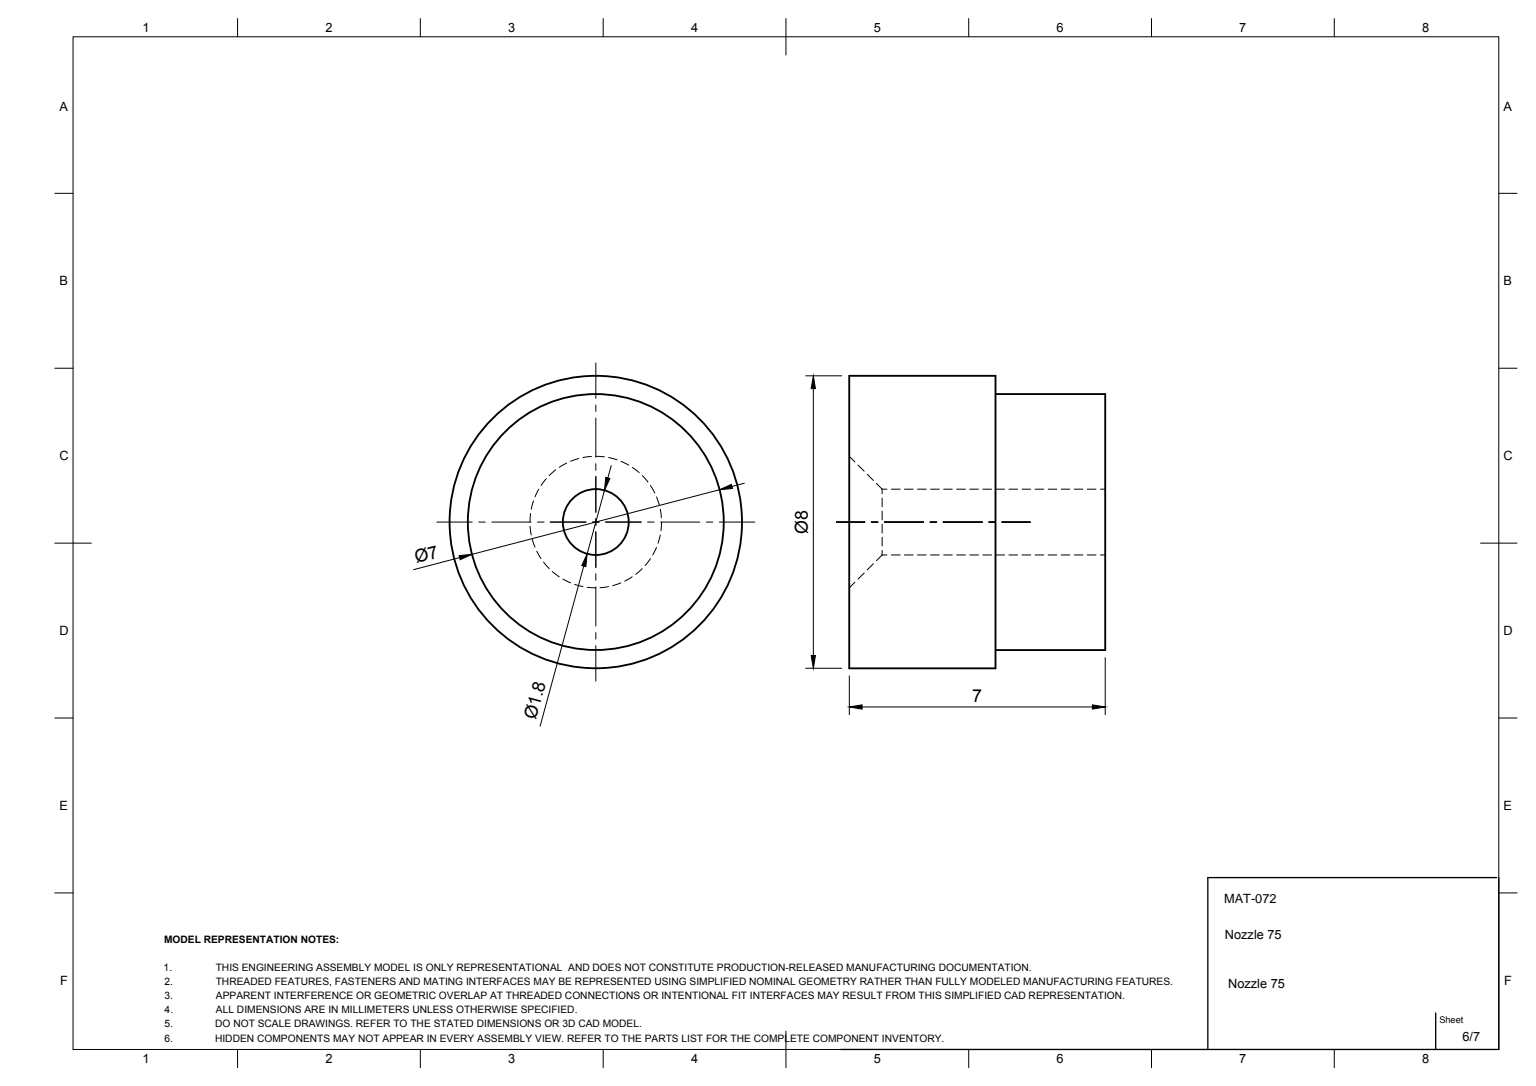
ISO-10303-21;
HEADER;
/* Generated by software containing ST-Developer
 * from STEP Tools, Inc. (www.steptools.com) 
 */

FILE_DESCRIPTION(
/* description */ (''),
/* implementation_level */ '2;1');

FILE_NAME(
/* name */ 'Nozzle 75.step',
/* time_stamp */ '2026-10-24T10:30:45-07:00',
/* author */ (''),
/* organization */ (''),
/* preprocessor_version */ 'ST-DEVELOPER v20.2',
/* originating_system */ 'Autodesk Translation Framework v15.15.0.0',
/* authorisation */ '');

FILE_SCHEMA (('AUTOMOTIVE_DESIGN { 1 0 10303 214 3 1 1 }'));
ENDSEC;

DATA;
#10=MECHANICAL_DESIGN_GEOMETRIC_PRESENTATION_REPRESENTATION('',(#80),#5183);
#65=CONICAL_SURFACE('',#2646,1.80000000000001,0.785398163397454);
#70=SHAPE_REPRESENTATION_RELATIONSHIP('SRR','None',#5217,#75);
#75=ADVANCED_BREP_SHAPE_REPRESENTATION('',(#85),#5181);
#80=STYLED_ITEM('',(#5247),#85);
#85=MANIFOLD_SOLID_BREP('Nozzle 75',#2366);
#138=FACE_BOUND('',#588,.T.);
#139=FACE_BOUND('',#590,.T.);
#140=FACE_BOUND('',#594,.T.);
#200=PLANE('',#2639);
#201=PLANE('',#2641);
#202=PLANE('',#2647);
#398=FACE_OUTER_BOUND('',#586,.T.);
#399=FACE_OUTER_BOUND('',#587,.T.);
#400=FACE_OUTER_BOUND('',#589,.T.);
#401=FACE_OUTER_BOUND('',#591,.T.);
#402=FACE_OUTER_BOUND('',#592,.T.);
#403=FACE_OUTER_BOUND('',#593,.T.);
#404=FACE_OUTER_BOUND('',#595,.T.);
#586=EDGE_LOOP('',(#2108,#2109,#2110,#2111));
#587=EDGE_LOOP('',(#2112));
#588=EDGE_LOOP('',(#2113));
#589=EDGE_LOOP('',(#2114));
#590=EDGE_LOOP('',(#2115));
#591=EDGE_LOOP('',(#2116,#2117,#2118,#2119));
#592=EDGE_LOOP('',(#2120,#2121,#2122,#2123));
#593=EDGE_LOOP('',(#2124));
#594=EDGE_LOOP('',(#2125));
#595=EDGE_LOOP('',(#2126,#2127,#2128,#2129));
#690=CIRCLE('',#2637,4.);
#691=CIRCLE('',#2638,4.);
#692=CIRCLE('',#2640,3.49999999999993);
#693=CIRCLE('',#2642,1.80000000000001);
#694=CIRCLE('',#2644,0.900000000000014);
#695=CIRCLE('',#2645,0.899999999999985);
#696=CIRCLE('',#2648,3.49999999999993);
#846=LINE('',#5110,#996);
#847=LINE('',#5122,#997);
#848=LINE('',#5125,#998);
#849=LINE('',#5130,#999);
#996=VECTOR('',#3248,4.);
#997=VECTOR('',#3263,0.899999999999989);
#998=VECTOR('',#3268,1.80000000000001);
#999=VECTOR('',#3275,3.49999999999992);
#1196=VERTEX_POINT('',#5107);
#1197=VERTEX_POINT('',#5109);
#1198=VERTEX_POINT('',#5113);
#1199=VERTEX_POINT('',#5116);
#1200=VERTEX_POINT('',#5119);
#1201=VERTEX_POINT('',#5121);
#1202=VERTEX_POINT('',#5127);
#1502=EDGE_CURVE('',#1196,#1196,#690,.T.);
#1503=EDGE_CURVE('',#1196,#1197,#846,.T.);
#1504=EDGE_CURVE('',#1197,#1197,#691,.T.);
#1505=EDGE_CURVE('',#1198,#1198,#692,.T.);
#1506=EDGE_CURVE('',#1199,#1199,#693,.T.);
#1507=EDGE_CURVE('',#1200,#1200,#694,.T.);
#1508=EDGE_CURVE('',#1200,#1201,#847,.T.);
#1509=EDGE_CURVE('',#1201,#1201,#695,.T.);
#1510=EDGE_CURVE('',#1201,#1199,#848,.T.);
#1511=EDGE_CURVE('',#1202,#1202,#696,.T.);
#1512=EDGE_CURVE('',#1198,#1202,#849,.T.);
#2108=ORIENTED_EDGE('',*,*,#1502,.T.);
#2109=ORIENTED_EDGE('',*,*,#1503,.T.);
#2110=ORIENTED_EDGE('',*,*,#1504,.F.);
#2111=ORIENTED_EDGE('',*,*,#1503,.F.);
#2112=ORIENTED_EDGE('',*,*,#1504,.T.);
#2113=ORIENTED_EDGE('',*,*,#1505,.F.);
#2114=ORIENTED_EDGE('',*,*,#1502,.F.);
#2115=ORIENTED_EDGE('',*,*,#1506,.F.);
#2116=ORIENTED_EDGE('',*,*,#1507,.T.);
#2117=ORIENTED_EDGE('',*,*,#1508,.T.);
#2118=ORIENTED_EDGE('',*,*,#1509,.T.);
#2119=ORIENTED_EDGE('',*,*,#1508,.F.);
#2120=ORIENTED_EDGE('',*,*,#1509,.F.);
#2121=ORIENTED_EDGE('',*,*,#1510,.T.);
#2122=ORIENTED_EDGE('',*,*,#1506,.T.);
#2123=ORIENTED_EDGE('',*,*,#1510,.F.);
#2124=ORIENTED_EDGE('',*,*,#1511,.T.);
#2125=ORIENTED_EDGE('',*,*,#1507,.F.);
#2126=ORIENTED_EDGE('',*,*,#1505,.T.);
#2127=ORIENTED_EDGE('',*,*,#1512,.T.);
#2128=ORIENTED_EDGE('',*,*,#1511,.F.);
#2129=ORIENTED_EDGE('',*,*,#1512,.F.);
#2217=CYLINDRICAL_SURFACE('',#2636,4.);
#2218=CYLINDRICAL_SURFACE('',#2643,0.899999999999989);
#2219=CYLINDRICAL_SURFACE('',#2649,3.49999999999993);
#2349=ADVANCED_FACE('',(#398),#2217,.T.);
#2350=ADVANCED_FACE('',(#399,#138),#200,.T.);
#2351=ADVANCED_FACE('',(#400,#139),#201,.F.);
#2352=ADVANCED_FACE('',(#401),#2218,.F.);
#2353=ADVANCED_FACE('',(#402),#65,.F.);
#2354=ADVANCED_FACE('',(#403,#140),#202,.T.);
#2355=ADVANCED_FACE('',(#404),#2219,.T.);
#2366=CLOSED_SHELL('',(#2349,#2350,#2351,#2352,#2353,#2354,#2355));
#2635=AXIS2_PLACEMENT_3D('',#5105,#3242,#3243);
#2636=AXIS2_PLACEMENT_3D('',#5106,#3244,#3245);
#2637=AXIS2_PLACEMENT_3D('',#5108,#3246,#3247);
#2638=AXIS2_PLACEMENT_3D('',#5111,#3249,#3250);
#2639=AXIS2_PLACEMENT_3D('',#5112,#3251,#3252);
#2640=AXIS2_PLACEMENT_3D('',#5114,#3253,#3254);
#2641=AXIS2_PLACEMENT_3D('',#5115,#3255,#3256);
#2642=AXIS2_PLACEMENT_3D('',#5117,#3257,#3258);
#2643=AXIS2_PLACEMENT_3D('',#5118,#3259,#3260);
#2644=AXIS2_PLACEMENT_3D('',#5120,#3261,#3262);
#2645=AXIS2_PLACEMENT_3D('',#5123,#3264,#3265);
#2646=AXIS2_PLACEMENT_3D('',#5124,#3266,#3267);
#2647=AXIS2_PLACEMENT_3D('',#5126,#3269,#3270);
#2648=AXIS2_PLACEMENT_3D('',#5128,#3271,#3272);
#2649=AXIS2_PLACEMENT_3D('',#5129,#3273,#3274);
#3242=DIRECTION('axis',(0.,0.,1.));
#3243=DIRECTION('refdir',(1.,0.,0.));
#3244=DIRECTION('center_axis',(-0.224143868042018,0.965925826289067,-0.129409522551263));
#3245=DIRECTION('ref_axis',(-0.974116947696296,-0.22604462437946,0.));
#3246=DIRECTION('center_axis',(0.224143868042018,-0.965925826289067,0.129409522551263));
#3247=DIRECTION('ref_axis',(0.974116947696296,0.22604462437946,0.));
#3248=DIRECTION('',(0.224143868042018,-0.965925826289067,0.129409522551263));
#3249=DIRECTION('center_axis',(0.224143868042018,-0.965925826289067,0.129409522551263));
#3250=DIRECTION('ref_axis',(0.974116947696296,0.22604462437946,0.));
#3251=DIRECTION('center_axis',(0.224143868042018,-0.965925826289067,0.129409522551263));
#3252=DIRECTION('ref_axis',(0.,-0.132788176096111,-0.991144439670156));
#3253=DIRECTION('center_axis',(0.224143868042018,-0.965925826289067,0.129409522551263));
#3254=DIRECTION('ref_axis',(0.974116947696296,0.22604462437946,0.));
#3255=DIRECTION('center_axis',(0.224143868042018,-0.965925826289067,0.129409522551263));
#3256=DIRECTION('ref_axis',(0.,-0.132788176096111,-0.991144439670156));
#3257=DIRECTION('center_axis',(-0.224143868042018,0.965925826289067,-0.129409522551263));
#3258=DIRECTION('ref_axis',(-0.974116947696296,-0.22604462437946,0.));
#3259=DIRECTION('center_axis',(-0.224143868042018,0.965925826289067,-0.129409522551263));
#3260=DIRECTION('ref_axis',(-0.974116947696296,-0.22604462437946,0.));
#3261=DIRECTION('center_axis',(0.224143868042018,-0.965925826289067,0.129409522551263));
#3262=DIRECTION('ref_axis',(0.974116947696296,0.22604462437946,0.));
#3263=DIRECTION('',(-0.224143868042018,0.965925826289067,-0.129409522551263));
#3264=DIRECTION('center_axis',(-0.224143868042018,0.965925826289067,-0.129409522551263));
#3265=DIRECTION('ref_axis',(-0.974116947696296,-0.22604462437946,0.));
#3266=DIRECTION('center_axis',(-0.224143868042018,0.965925826289067,-0.129409522551263));
#3267=DIRECTION('ref_axis',(-0.974116947696296,-0.22604462437946,0.));
#3268=DIRECTION('',(0.530311050330904,0.842850388641698,-0.091506350946111));
#3269=DIRECTION('center_axis',(0.224143868042018,-0.965925826289067,0.129409522551263));
#3270=DIRECTION('ref_axis',(0.,-0.132788176096111,-0.991144439670156));
#3271=DIRECTION('center_axis',(0.224143868042018,-0.965925826289067,0.129409522551263));
#3272=DIRECTION('ref_axis',(0.974116947696296,0.22604462437946,0.));
#3273=DIRECTION('center_axis',(-0.224143868042018,0.965925826289067,-0.129409522551263));
#3274=DIRECTION('ref_axis',(-0.974116947696296,-0.22604462437946,0.));
#3275=DIRECTION('',(0.224143868042018,-0.965925826289067,0.129409522551263));
#5105=CARTESIAN_POINT('',(0.,0.,0.));
#5106=CARTESIAN_POINT('Origin',(-88.8998569762207,131.101020514434,-63.3263563561378));
#5107=CARTESIAN_POINT('',(-85.8999646576036,135.868902317108,-63.8439944463428));
#5108=CARTESIAN_POINT('Origin',(-89.7964324483888,134.96472381959,-63.8439944463428));
#5109=CARTESIAN_POINT('',(-85.0033891854356,132.005199011951,-63.3263563561378));
#5110=CARTESIAN_POINT('',(-85.0033891854356,132.005199011951,-63.3263563561378));
#5111=CARTESIAN_POINT('Origin',(-88.8998569762207,131.101020514434,-63.3263563561378));
#5112=CARTESIAN_POINT('Origin',(-88.8998569762207,131.101020514434,-63.3263563561378));
#5113=CARTESIAN_POINT('',(-85.4904476592837,131.892176699762,-63.3263563561378));
#5114=CARTESIAN_POINT('Origin',(-88.8998569762207,131.101020514434,-63.3263563561378));
#5115=CARTESIAN_POINT('Origin',(-89.7964324483888,134.96472381959,-63.8439944463428));
#5116=CARTESIAN_POINT('',(-88.0430219425354,135.371604143473,-63.8439944463428));
#5117=CARTESIAN_POINT('Origin',(-89.7964324483888,134.96472381959,-63.8439944463428));
#5118=CARTESIAN_POINT('Origin',(-89.7964324483888,134.96472381959,-63.8439944463428));
#5119=CARTESIAN_POINT('',(-87.350720119168,128.406683197508,-62.938127788484));
#5120=CARTESIAN_POINT('Origin',(-88.2274253720946,128.203243035566,-62.938127788484));
#5121=CARTESIAN_POINT('',(-88.7179977142243,134.298830737871,-63.7275258760467));
#5122=CARTESIAN_POINT('',(-88.9197271954621,135.168163981531,-63.8439944463428));
#5123=CARTESIAN_POINT('Origin',(-89.5947029671509,134.09539057593,-63.7275258760467));
#5124=CARTESIAN_POINT('Origin',(-89.7964324483888,134.96472381959,-63.8439944463428));
#5125=CARTESIAN_POINT('',(-88.0430219425354,135.371604143473,-63.8439944463428));
#5126=CARTESIAN_POINT('Origin',(-88.2274253720946,128.203243035566,-62.938127788484));
#5127=CARTESIAN_POINT('',(-84.8180160551577,128.994399220895,-62.938127788484));
#5128=CARTESIAN_POINT('Origin',(-88.2274253720946,128.203243035566,-62.938127788484));
#5129=CARTESIAN_POINT('Origin',(-88.2274253720946,128.203243035566,-62.938127788484));
#5130=CARTESIAN_POINT('',(-84.8180160551577,128.994399220895,-62.938127788484));
#5174=UNCERTAINTY_MEASURE_WITH_UNIT(LENGTH_MEASURE(0.01),#5184,
'DISTANCE_ACCURACY_VALUE',
'Maximum model space distance between geometric entities at asserted c
onnectivities');
#5176=UNCERTAINTY_MEASURE_WITH_UNIT(LENGTH_MEASURE(0.01),#5184,
'DISTANCE_ACCURACY_VALUE',
'Maximum model space distance between geometric entities at asserted c
onnectivities');
#5181=(
GEOMETRIC_REPRESENTATION_CONTEXT(3)
GLOBAL_UNCERTAINTY_ASSIGNED_CONTEXT((#5174))
GLOBAL_UNIT_ASSIGNED_CONTEXT((#5184,#5186,#5187))
REPRESENTATION_CONTEXT('','3D')
);
#5183=(
GEOMETRIC_REPRESENTATION_CONTEXT(3)
GLOBAL_UNCERTAINTY_ASSIGNED_CONTEXT((#5176))
GLOBAL_UNIT_ASSIGNED_CONTEXT((#5184,#5186,#5187))
REPRESENTATION_CONTEXT('','3D')
);
#5184=(
LENGTH_UNIT()
NAMED_UNIT(*)
SI_UNIT(.MILLI.,.METRE.)
);
#5186=(
NAMED_UNIT(*)
PLANE_ANGLE_UNIT()
SI_UNIT($,.RADIAN.)
);
#5187=(
NAMED_UNIT(*)
SI_UNIT($,.STERADIAN.)
SOLID_ANGLE_UNIT()
);
#5192=SHAPE_DEFINITION_REPRESENTATION(#5198,#5217);
#5198=PRODUCT_DEFINITION_SHAPE('',$,#5224);
#5217=SHAPE_REPRESENTATION('',(#2635),#5181);
#5219=PRODUCT_DEFINITION_CONTEXT('part definition',#5239,'design');
#5224=PRODUCT_DEFINITION('Nozzle 75','Nozzle 75',#5230,#5219);
#5230=PRODUCT_DEFINITION_FORMATION('',$,#5245);
#5239=APPLICATION_CONTEXT(
'Core Data for Automotive Mechanical Design Process');
#5240=PRODUCT_CONTEXT('part definition',#5239,'mechanical');
#5245=PRODUCT('Nozzle 75','Nozzle 75',$,(#5240));
#5247=PRESENTATION_STYLE_ASSIGNMENT((#5248));
#5248=SURFACE_STYLE_USAGE(.BOTH.,#5249);
#5249=SURFACE_SIDE_STYLE('',(#5250));
#5250=SURFACE_STYLE_FILL_AREA(#5251);
#5251=FILL_AREA_STYLE('Steel - Satin',(#5252));
#5252=FILL_AREA_STYLE_COLOUR('Steel - Satin',#5253);
#5253=COLOUR_RGB('Steel - Satin',0.627450980392157,0.627450980392157,0.627450980392157);
ENDSEC;
END-ISO-10303-21;
